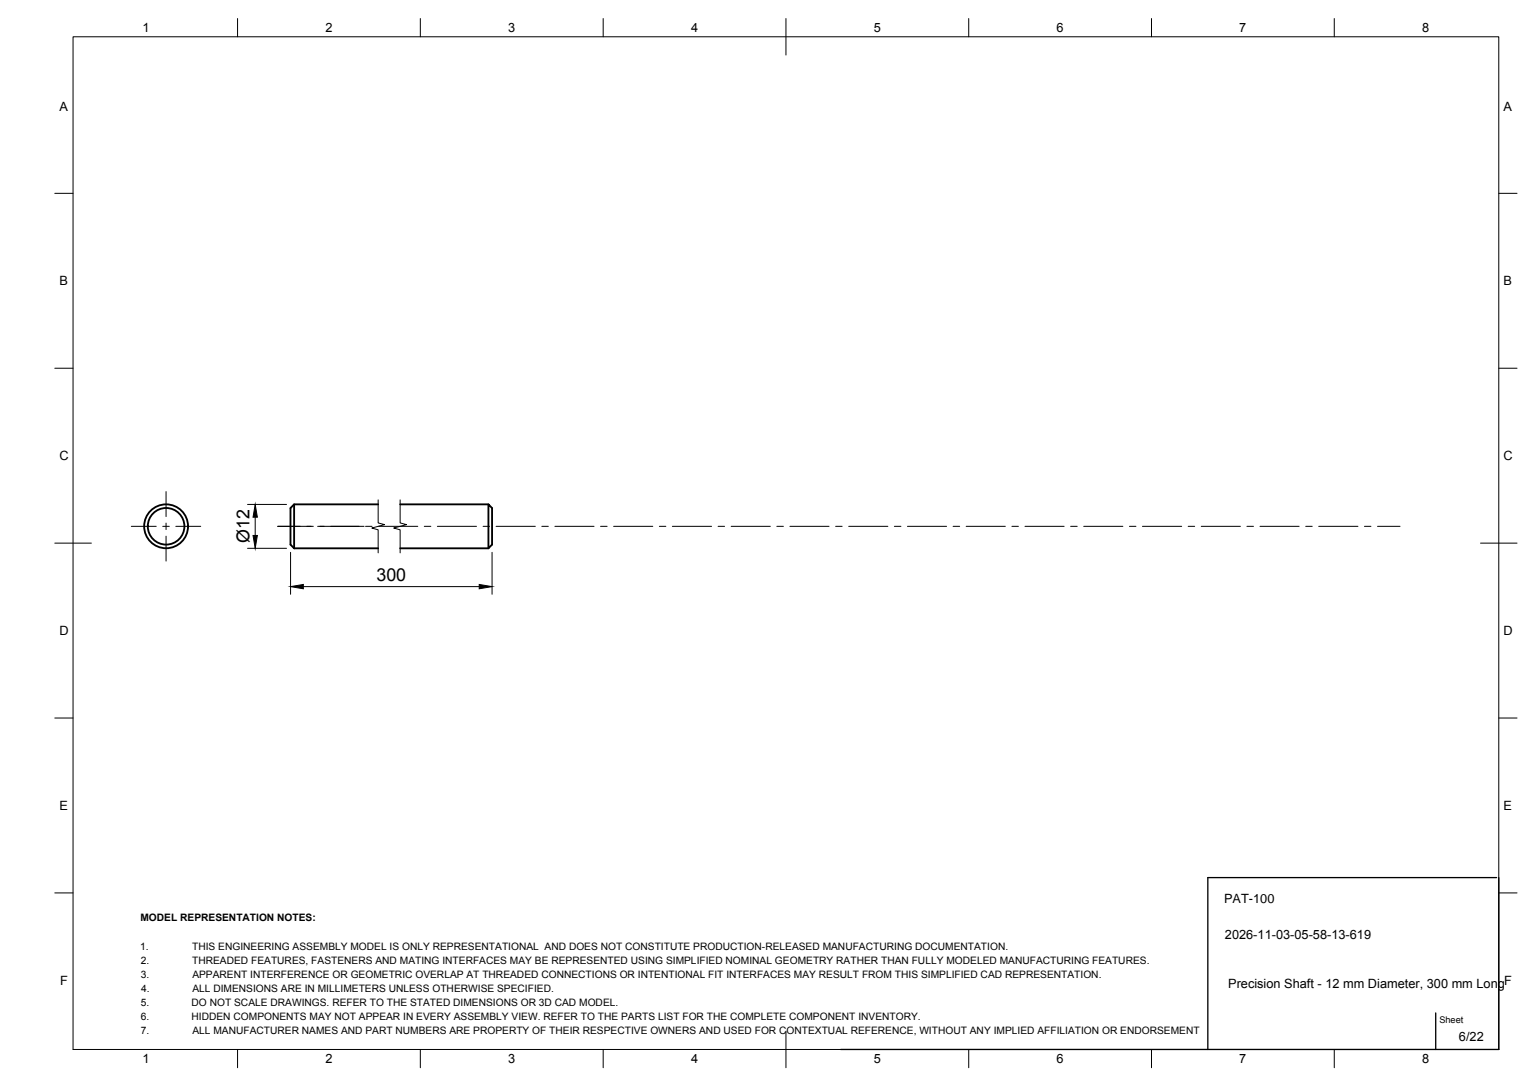
ISO-10303-21;
HEADER;
/* Generated by software containing ST-Developer
 * from STEP Tools, Inc. (www.steptools.com) 
 */

FILE_DESCRIPTION(
/* description */ (''),
/* implementation_level */ '2;1');

FILE_NAME(
/* name */ 'Precision Shaft - 12 mm Diameter, 300 mm Long.step',
/* time_stamp */ '2026-10-29T16:43:51-07:00',
/* author */ (''),
/* organization */ (''),
/* preprocessor_version */ 'ST-DEVELOPER v20.2',
/* originating_system */ 'Autodesk Translation Framework v15.17.0.0',
/* authorisation */ '');

FILE_SCHEMA (('AUTOMOTIVE_DESIGN { 1 0 10303 214 3 1 1 }'));
ENDSEC;

DATA;
#10=MECHANICAL_DESIGN_GEOMETRIC_PRESENTATION_REPRESENTATION('',(#366),#10292);
#293=CONICAL_SURFACE('',#5347,0.55,0.785398163397448);
#294=CONICAL_SURFACE('',#5353,0.55,0.785398163397441);
#320=SHAPE_REPRESENTATION_RELATIONSHIP('SRR','None',#10416,#343);
#343=ADVANCED_BREP_SHAPE_REPRESENTATION('',(#389),#10268);
#366=STYLED_ITEM('',(#10628),#389);
#389=MANIFOLD_SOLID_BREP('Body1',#5008);
#537=PLANE('',#5352);
#538=PLANE('',#5355);
#732=FACE_OUTER_BOUND('',#1052,.T.);
#733=FACE_OUTER_BOUND('',#1053,.T.);
#734=FACE_OUTER_BOUND('',#1054,.T.);
#735=FACE_OUTER_BOUND('',#1055,.T.);
#736=FACE_OUTER_BOUND('',#1056,.T.);
#1052=EDGE_LOOP('',(#3529,#3530,#3531,#3532));
#1053=EDGE_LOOP('',(#3533,#3534,#3535,#3536));
#1054=EDGE_LOOP('',(#3537));
#1055=EDGE_LOOP('',(#3538,#3539,#3540,#3541));
#1056=EDGE_LOOP('',(#3542));
#1439=LINE('',#7536,#1831);
#1440=LINE('',#7541,#1832);
#1441=LINE('',#7546,#1833);
#1831=VECTOR('',#6012,0.55);
#1832=VECTOR('',#6019,0.6);
#1833=VECTOR('',#6026,0.55);
#2227=CIRCLE('',#5348,0.6);
#2228=CIRCLE('',#5349,0.5);
#2229=CIRCLE('',#5351,0.6);
#2230=CIRCLE('',#5354,0.5);
#2434=VERTEX_POINT('',#7533);
#2435=VERTEX_POINT('',#7535);
#2436=VERTEX_POINT('',#7539);
#2437=VERTEX_POINT('',#7544);
#2855=EDGE_CURVE('',#2434,#2434,#2227,.T.);
#2856=EDGE_CURVE('',#2434,#2435,#1439,.T.);
#2857=EDGE_CURVE('',#2435,#2435,#2228,.T.);
#2858=EDGE_CURVE('',#2436,#2436,#2229,.T.);
#2859=EDGE_CURVE('',#2436,#2434,#1440,.T.);
#2860=EDGE_CURVE('',#2437,#2437,#2230,.T.);
#2861=EDGE_CURVE('',#2437,#2436,#1441,.T.);
#3529=ORIENTED_EDGE('',*,*,#2855,.T.);
#3530=ORIENTED_EDGE('',*,*,#2856,.T.);
#3531=ORIENTED_EDGE('',*,*,#2857,.T.);
#3532=ORIENTED_EDGE('',*,*,#2856,.F.);
#3533=ORIENTED_EDGE('',*,*,#2858,.F.);
#3534=ORIENTED_EDGE('',*,*,#2859,.T.);
#3535=ORIENTED_EDGE('',*,*,#2855,.F.);
#3536=ORIENTED_EDGE('',*,*,#2859,.F.);
#3537=ORIENTED_EDGE('',*,*,#2857,.F.);
#3538=ORIENTED_EDGE('',*,*,#2860,.T.);
#3539=ORIENTED_EDGE('',*,*,#2861,.T.);
#3540=ORIENTED_EDGE('',*,*,#2858,.T.);
#3541=ORIENTED_EDGE('',*,*,#2861,.F.);
#3542=ORIENTED_EDGE('',*,*,#2860,.F.);
#4653=CYLINDRICAL_SURFACE('',#5350,0.6);
#4741=ADVANCED_FACE('',(#732),#293,.T.);
#4742=ADVANCED_FACE('',(#733),#4653,.T.);
#4743=ADVANCED_FACE('',(#734),#537,.F.);
#4744=ADVANCED_FACE('',(#735),#294,.T.);
#4745=ADVANCED_FACE('',(#736),#538,.T.);
#5008=CLOSED_SHELL('',(#4741,#4742,#4743,#4744,#4745));
#5346=AXIS2_PLACEMENT_3D('',#7531,#6006,#6007);
#5347=AXIS2_PLACEMENT_3D('',#7532,#6008,#6009);
#5348=AXIS2_PLACEMENT_3D('',#7534,#6010,#6011);
#5349=AXIS2_PLACEMENT_3D('',#7537,#6013,#6014);
#5350=AXIS2_PLACEMENT_3D('',#7538,#6015,#6016);
#5351=AXIS2_PLACEMENT_3D('',#7540,#6017,#6018);
#5352=AXIS2_PLACEMENT_3D('',#7542,#6020,#6021);
#5353=AXIS2_PLACEMENT_3D('',#7543,#6022,#6023);
#5354=AXIS2_PLACEMENT_3D('',#7545,#6024,#6025);
#5355=AXIS2_PLACEMENT_3D('',#7547,#6027,#6028);
#6006=DIRECTION('axis',(0.,0.,1.));
#6007=DIRECTION('refdir',(1.,0.,0.));
#6008=DIRECTION('center_axis',(1.,0.,0.));
#6009=DIRECTION('ref_axis',(0.,0.,-1.));
#6010=DIRECTION('center_axis',(-1.,0.,0.));
#6011=DIRECTION('ref_axis',(0.,0.,-1.));
#6012=DIRECTION('',(-0.707106781186548,8.65956056235493E-17,-0.707106781186547));
#6013=DIRECTION('center_axis',(1.,0.,0.));
#6014=DIRECTION('ref_axis',(0.,0.,-1.));
#6015=DIRECTION('center_axis',(1.,0.,0.));
#6016=DIRECTION('ref_axis',(0.,0.,-1.));
#6017=DIRECTION('center_axis',(1.,0.,0.));
#6018=DIRECTION('ref_axis',(0.,0.,-1.));
#6019=DIRECTION('',(-1.,0.,0.));
#6020=DIRECTION('center_axis',(1.,0.,0.));
#6021=DIRECTION('ref_axis',(0.,0.,-1.));
#6022=DIRECTION('center_axis',(-1.,0.,0.));
#6023=DIRECTION('ref_axis',(0.,0.,-1.));
#6024=DIRECTION('center_axis',(-1.,0.,0.));
#6025=DIRECTION('ref_axis',(0.,0.,-1.));
#6026=DIRECTION('',(-0.707106781186553,-8.65956056235487E-17,0.707106781186542));
#6027=DIRECTION('center_axis',(1.,0.,0.));
#6028=DIRECTION('ref_axis',(0.,0.,-1.));
#7531=CARTESIAN_POINT('',(0.,0.,0.));
#7532=CARTESIAN_POINT('Origin',(0.05,0.,0.));
#7533=CARTESIAN_POINT('',(0.1,7.34788079488412E-17,0.6));
#7534=CARTESIAN_POINT('Origin',(0.1,0.,0.));
#7535=CARTESIAN_POINT('',(0.,-6.12323399573677E-17,0.5));
#7536=CARTESIAN_POINT('',(0.05,-6.73555739531044E-17,0.55));
#7537=CARTESIAN_POINT('Origin',(0.,0.,0.));
#7538=CARTESIAN_POINT('Origin',(0.,0.,0.));
#7539=CARTESIAN_POINT('',(29.9,-7.34788079488412E-17,0.6));
#7540=CARTESIAN_POINT('Origin',(29.9,0.,0.));
#7541=CARTESIAN_POINT('',(0.,-7.34788079488412E-17,0.6));
#7542=CARTESIAN_POINT('Origin',(0.,0.,0.));
#7543=CARTESIAN_POINT('Origin',(29.95,0.,0.));
#7544=CARTESIAN_POINT('',(30.,6.12323399573677E-17,0.5));
#7545=CARTESIAN_POINT('Origin',(30.,0.,0.));
#7546=CARTESIAN_POINT('',(29.95,-6.73555739531044E-17,0.55));
#7547=CARTESIAN_POINT('Origin',(30.,0.,0.));
#10240=UNCERTAINTY_MEASURE_WITH_UNIT(LENGTH_MEASURE(0.001),#10293,
'DISTANCE_ACCURACY_VALUE',
'Maximum model space distance between geometric entities at asserted c
onnectivities');
#10264=UNCERTAINTY_MEASURE_WITH_UNIT(LENGTH_MEASURE(0.001),#10293,
'DISTANCE_ACCURACY_VALUE',
'Maximum model space distance between geometric entities at asserted c
onnectivities');
#10268=(
GEOMETRIC_REPRESENTATION_CONTEXT(3)
GLOBAL_UNCERTAINTY_ASSIGNED_CONTEXT((#10240))
GLOBAL_UNIT_ASSIGNED_CONTEXT((#10293,#10295,#10296))
REPRESENTATION_CONTEXT('','3D')
);
#10292=(
GEOMETRIC_REPRESENTATION_CONTEXT(3)
GLOBAL_UNCERTAINTY_ASSIGNED_CONTEXT((#10264))
GLOBAL_UNIT_ASSIGNED_CONTEXT((#10293,#10295,#10296))
REPRESENTATION_CONTEXT('','3D')
);
#10293=(
LENGTH_UNIT()
NAMED_UNIT(*)
SI_UNIT(.CENTI.,.METRE.)
);
#10295=(
NAMED_UNIT(*)
PLANE_ANGLE_UNIT()
SI_UNIT($,.RADIAN.)
);
#10296=(
NAMED_UNIT(*)
SI_UNIT($,.STERADIAN.)
SOLID_ANGLE_UNIT()
);
#10300=SHAPE_DEFINITION_REPRESENTATION(#10327,#10416);
#10327=PRODUCT_DEFINITION_SHAPE('',$,#10444);
#10416=SHAPE_REPRESENTATION('',(#5346),#10268);
#10440=PRODUCT_DEFINITION_CONTEXT('part definition',#10523,'design');
#10444=PRODUCT_DEFINITION('Precision Shaft - 12 mm Diameter, 300 mm Long',
'Precision Shaft - 12 mm Diameter, 300 mm Long',#10471,#10440);
#10471=PRODUCT_DEFINITION_FORMATION('',$,#10528);
#10523=APPLICATION_CONTEXT(
'Core Data for Automotive Mechanical Design Process');
#10524=PRODUCT_CONTEXT('part definition',#10523,'mechanical');
#10528=PRODUCT('Precision Shaft - 12 mm Diameter, 300 mm Long',
'Precision Shaft - 12 mm Diameter, 300 mm Long',
'Precision Shaft - 12 mm Diameter, 300 mm Long',(#10524));
#10622=COLOUR_RGB('Grey',0.48,0.52,0.57);
#10623=FILL_AREA_STYLE_COLOUR('',#10622);
#10624=FILL_AREA_STYLE('',(#10623));
#10625=SURFACE_STYLE_FILL_AREA(#10624);
#10626=SURFACE_SIDE_STYLE('',(#10625));
#10627=SURFACE_STYLE_USAGE(.BOTH.,#10626);
#10628=PRESENTATION_STYLE_ASSIGNMENT((#10627));
ENDSEC;
END-ISO-10303-21;
